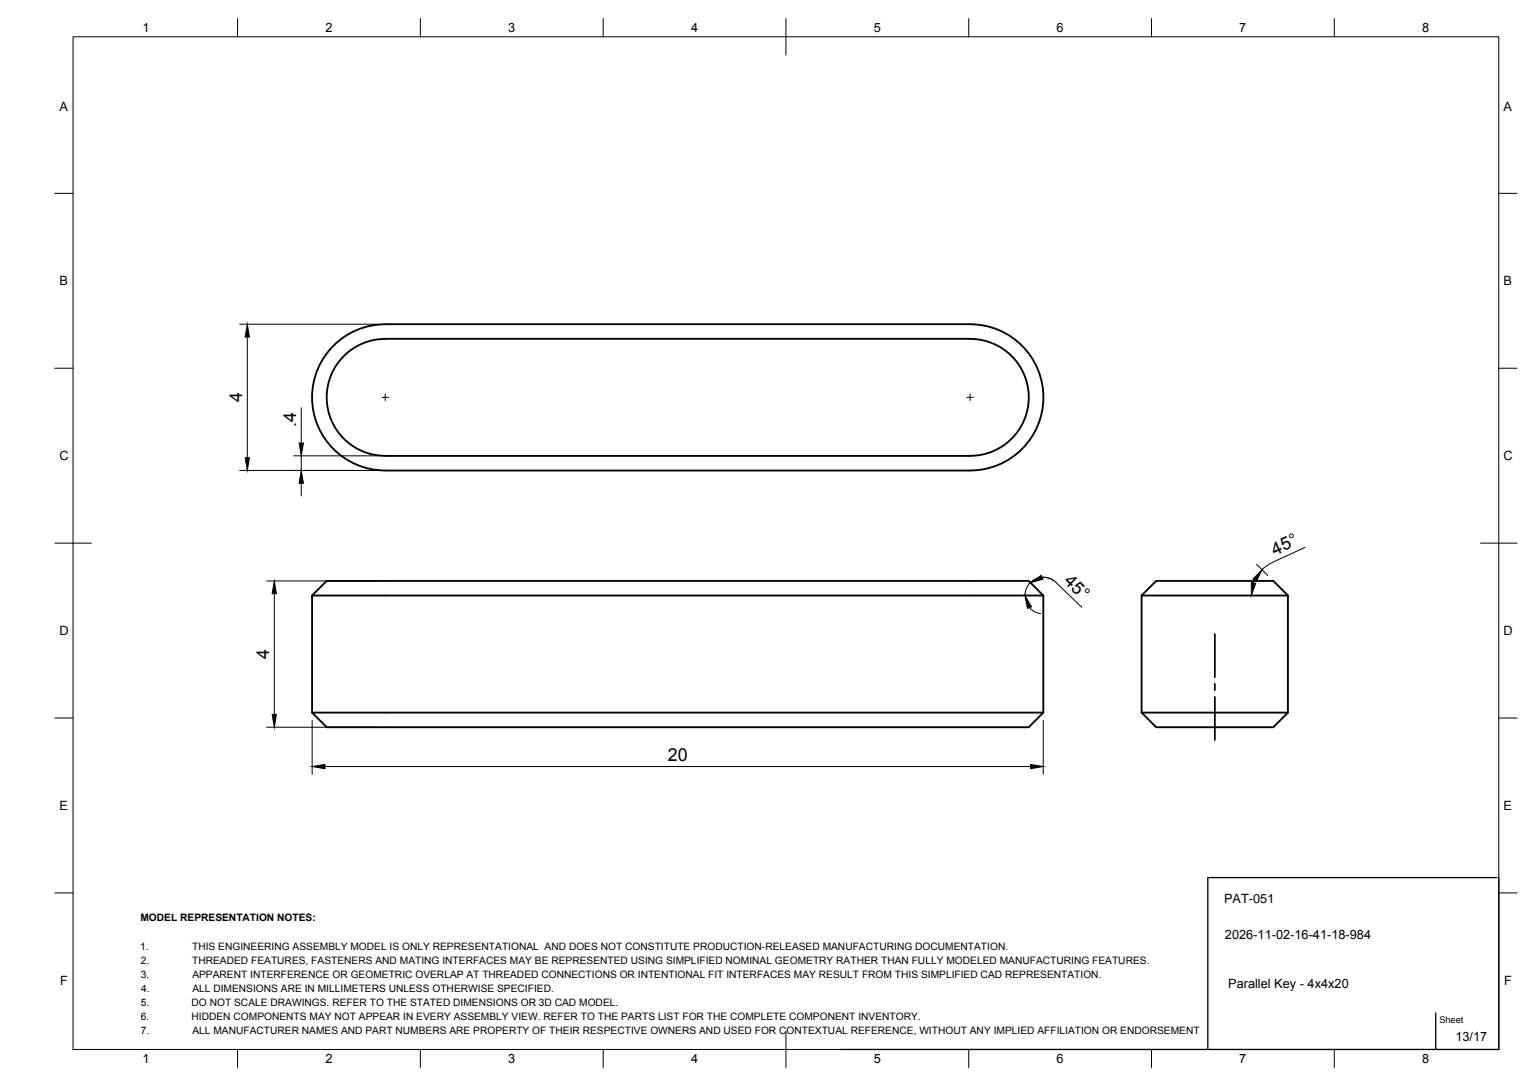
ISO-10303-21;
HEADER;
/* Generated by software containing ST-Developer
 * from STEP Tools, Inc. (www.steptools.com) 
 */

FILE_DESCRIPTION(
/* description */ ('Hand-crank flanged shaft unit'),
/* implementation_level */ '2;1');

FILE_NAME(
/* name */ 'Parallel Key - 4x4x20.step',
/* time_stamp */ '2026-10-27T18:35:45-07:00',
/* author */ (''),
/* organization */ (''),
/* preprocessor_version */ 'ST-DEVELOPER v20.2',
/* originating_system */ 'Autodesk Translation Framework v15.17.0.0',
/* authorisation */ '');

FILE_SCHEMA (('AUTOMOTIVE_DESIGN { 1 0 10303 214 3 1 1 }'));
ENDSEC;

DATA;
#10=MECHANICAL_DESIGN_GEOMETRIC_PRESENTATION_REPRESENTATION('',(#296),#6805);
#18=CONICAL_SURFACE('',#3857,0.18,0.785398163397448);
#19=CONICAL_SURFACE('',#3861,0.18,0.785398163397448);
#20=CONICAL_SURFACE('',#3869,0.18,0.785398163397449);
#21=CONICAL_SURFACE('',#3872,0.18,0.785398163397449);
#255=SHAPE_REPRESENTATION_RELATIONSHIP('SRR','None',#6918,#275);
#275=ADVANCED_BREP_SHAPE_REPRESENTATION('',(#316),#6801);
#296=STYLED_ITEM('',(#7091),#316);
#316=MANIFOLD_SOLID_BREP('Body1',#3338);
#487=PLANE('',#3856);
#488=PLANE('',#3860);
#489=PLANE('',#3866);
#490=PLANE('',#3867);
#491=PLANE('',#3868);
#492=PLANE('',#3871);
#493=PLANE('',#3876);
#494=PLANE('',#3877);
#658=FACE_OUTER_BOUND('',#930,.T.);
#659=FACE_OUTER_BOUND('',#931,.T.);
#660=FACE_OUTER_BOUND('',#932,.T.);
#661=FACE_OUTER_BOUND('',#933,.T.);
#662=FACE_OUTER_BOUND('',#934,.T.);
#663=FACE_OUTER_BOUND('',#935,.T.);
#664=FACE_OUTER_BOUND('',#936,.T.);
#665=FACE_OUTER_BOUND('',#937,.T.);
#666=FACE_OUTER_BOUND('',#938,.T.);
#667=FACE_OUTER_BOUND('',#939,.T.);
#668=FACE_OUTER_BOUND('',#940,.T.);
#669=FACE_OUTER_BOUND('',#941,.T.);
#670=FACE_OUTER_BOUND('',#942,.T.);
#671=FACE_OUTER_BOUND('',#943,.T.);
#930=EDGE_LOOP('',(#2885,#2886,#2887,#2888));
#931=EDGE_LOOP('',(#2889,#2890,#2891,#2892));
#932=EDGE_LOOP('',(#2893,#2894,#2895,#2896));
#933=EDGE_LOOP('',(#2897,#2898,#2899,#2900));
#934=EDGE_LOOP('',(#2901,#2902,#2903,#2904));
#935=EDGE_LOOP('',(#2905,#2906,#2907,#2908));
#936=EDGE_LOOP('',(#2909,#2910,#2911,#2912));
#937=EDGE_LOOP('',(#2913,#2914,#2915,#2916));
#938=EDGE_LOOP('',(#2917,#2918,#2919,#2920));
#939=EDGE_LOOP('',(#2921,#2922,#2923,#2924));
#940=EDGE_LOOP('',(#2925,#2926,#2927,#2928));
#941=EDGE_LOOP('',(#2929,#2930,#2931,#2932));
#942=EDGE_LOOP('',(#2933,#2934,#2935,#2936));
#943=EDGE_LOOP('',(#2937,#2938,#2939,#2940));
#1142=LINE('',#6488,#1370);
#1143=LINE('',#6490,#1371);
#1144=LINE('',#6492,#1372);
#1145=LINE('',#6493,#1373);
#1146=LINE('',#6497,#1374);
#1147=LINE('',#6503,#1375);
#1148=LINE('',#6504,#1376);
#1149=LINE('',#6505,#1377);
#1150=LINE('',#6511,#1378);
#1151=LINE('',#6514,#1379);
#1152=LINE('',#6517,#1380);
#1153=LINE('',#6518,#1381);
#1154=LINE('',#6522,#1382);
#1155=LINE('',#6524,#1383);
#1156=LINE('',#6525,#1384);
#1157=LINE('',#6528,#1385);
#1158=LINE('',#6533,#1386);
#1159=LINE('',#6534,#1387);
#1160=LINE('',#6535,#1388);
#1161=LINE('',#6540,#1389);
#1370=VECTOR('',#4707,1.);
#1371=VECTOR('',#4708,1.);
#1372=VECTOR('',#4709,1.);
#1373=VECTOR('',#4710,1.);
#1374=VECTOR('',#4713,1.);
#1375=VECTOR('',#4720,1.);
#1376=VECTOR('',#4721,1.);
#1377=VECTOR('',#4722,1.);
#1378=VECTOR('',#4731,1.);
#1379=VECTOR('',#4734,1.);
#1380=VECTOR('',#4737,1.);
#1381=VECTOR('',#4738,1.);
#1382=VECTOR('',#4743,1.);
#1383=VECTOR('',#4744,1.);
#1384=VECTOR('',#4745,1.);
#1385=VECTOR('',#4748,1.);
#1386=VECTOR('',#4753,1.);
#1387=VECTOR('',#4754,1.);
#1388=VECTOR('',#4755,1.);
#1389=VECTOR('',#4764,1.);
#1547=CIRCLE('',#3858,0.16);
#1548=CIRCLE('',#3859,0.2);
#1549=CIRCLE('',#3862,0.16);
#1550=CIRCLE('',#3863,0.2);
#1551=CIRCLE('',#3865,0.2);
#1552=CIRCLE('',#3870,0.16);
#1553=CIRCLE('',#3873,0.2);
#1554=CIRCLE('',#3874,0.16);
#1787=VERTEX_POINT('',#6486);
#1788=VERTEX_POINT('',#6487);
#1789=VERTEX_POINT('',#6489);
#1790=VERTEX_POINT('',#6491);
#1791=VERTEX_POINT('',#6495);
#1792=VERTEX_POINT('',#6496);
#1793=VERTEX_POINT('',#6501);
#1794=VERTEX_POINT('',#6502);
#1795=VERTEX_POINT('',#6510);
#1796=VERTEX_POINT('',#6512);
#1797=VERTEX_POINT('',#6516);
#1798=VERTEX_POINT('',#6521);
#1799=VERTEX_POINT('',#6523);
#1800=VERTEX_POINT('',#6527);
#1801=VERTEX_POINT('',#6531);
#1802=VERTEX_POINT('',#6532);
#2160=EDGE_CURVE('',#1787,#1788,#1142,.T.);
#2161=EDGE_CURVE('',#1788,#1789,#1143,.T.);
#2162=EDGE_CURVE('',#1789,#1790,#1144,.T.);
#2163=EDGE_CURVE('',#1790,#1787,#1145,.T.);
#2164=EDGE_CURVE('',#1791,#1792,#1146,.T.);
#2165=EDGE_CURVE('',#1792,#1788,#1547,.T.);
#2166=EDGE_CURVE('',#1787,#1791,#1548,.T.);
#2167=EDGE_CURVE('',#1793,#1794,#1147,.T.);
#2168=EDGE_CURVE('',#1794,#1792,#1148,.T.);
#2169=EDGE_CURVE('',#1791,#1793,#1149,.T.);
#2170=EDGE_CURVE('',#1789,#1794,#1549,.T.);
#2171=EDGE_CURVE('',#1793,#1790,#1550,.T.);
#2172=EDGE_CURVE('',#1795,#1787,#1150,.T.);
#2173=EDGE_CURVE('',#1796,#1795,#1551,.T.);
#2174=EDGE_CURVE('',#1796,#1791,#1151,.T.);
#2175=EDGE_CURVE('',#1797,#1790,#1152,.T.);
#2176=EDGE_CURVE('',#1795,#1797,#1153,.T.);
#2177=EDGE_CURVE('',#1798,#1795,#1154,.T.);
#2178=EDGE_CURVE('',#1797,#1799,#1155,.T.);
#2179=EDGE_CURVE('',#1799,#1798,#1156,.T.);
#2180=EDGE_CURVE('',#1800,#1796,#1157,.T.);
#2181=EDGE_CURVE('',#1798,#1800,#1552,.T.);
#2182=EDGE_CURVE('',#1801,#1802,#1158,.T.);
#2183=EDGE_CURVE('',#1802,#1796,#1159,.T.);
#2184=EDGE_CURVE('',#1800,#1801,#1160,.T.);
#2185=EDGE_CURVE('',#1797,#1802,#1553,.T.);
#2186=EDGE_CURVE('',#1801,#1799,#1554,.T.);
#2187=EDGE_CURVE('',#1802,#1793,#1161,.T.);
#2885=ORIENTED_EDGE('',*,*,#2160,.T.);
#2886=ORIENTED_EDGE('',*,*,#2161,.T.);
#2887=ORIENTED_EDGE('',*,*,#2162,.T.);
#2888=ORIENTED_EDGE('',*,*,#2163,.T.);
#2889=ORIENTED_EDGE('',*,*,#2164,.T.);
#2890=ORIENTED_EDGE('',*,*,#2165,.T.);
#2891=ORIENTED_EDGE('',*,*,#2160,.F.);
#2892=ORIENTED_EDGE('',*,*,#2166,.T.);
#2893=ORIENTED_EDGE('',*,*,#2167,.T.);
#2894=ORIENTED_EDGE('',*,*,#2168,.T.);
#2895=ORIENTED_EDGE('',*,*,#2164,.F.);
#2896=ORIENTED_EDGE('',*,*,#2169,.T.);
#2897=ORIENTED_EDGE('',*,*,#2162,.F.);
#2898=ORIENTED_EDGE('',*,*,#2170,.T.);
#2899=ORIENTED_EDGE('',*,*,#2167,.F.);
#2900=ORIENTED_EDGE('',*,*,#2171,.T.);
#2901=ORIENTED_EDGE('',*,*,#2166,.F.);
#2902=ORIENTED_EDGE('',*,*,#2172,.F.);
#2903=ORIENTED_EDGE('',*,*,#2173,.F.);
#2904=ORIENTED_EDGE('',*,*,#2174,.T.);
#2905=ORIENTED_EDGE('',*,*,#2163,.F.);
#2906=ORIENTED_EDGE('',*,*,#2175,.F.);
#2907=ORIENTED_EDGE('',*,*,#2176,.F.);
#2908=ORIENTED_EDGE('',*,*,#2172,.T.);
#2909=ORIENTED_EDGE('',*,*,#2161,.F.);
#2910=ORIENTED_EDGE('',*,*,#2165,.F.);
#2911=ORIENTED_EDGE('',*,*,#2168,.F.);
#2912=ORIENTED_EDGE('',*,*,#2170,.F.);
#2913=ORIENTED_EDGE('',*,*,#2177,.T.);
#2914=ORIENTED_EDGE('',*,*,#2176,.T.);
#2915=ORIENTED_EDGE('',*,*,#2178,.T.);
#2916=ORIENTED_EDGE('',*,*,#2179,.T.);
#2917=ORIENTED_EDGE('',*,*,#2180,.T.);
#2918=ORIENTED_EDGE('',*,*,#2173,.T.);
#2919=ORIENTED_EDGE('',*,*,#2177,.F.);
#2920=ORIENTED_EDGE('',*,*,#2181,.T.);
#2921=ORIENTED_EDGE('',*,*,#2182,.T.);
#2922=ORIENTED_EDGE('',*,*,#2183,.T.);
#2923=ORIENTED_EDGE('',*,*,#2180,.F.);
#2924=ORIENTED_EDGE('',*,*,#2184,.T.);
#2925=ORIENTED_EDGE('',*,*,#2178,.F.);
#2926=ORIENTED_EDGE('',*,*,#2185,.T.);
#2927=ORIENTED_EDGE('',*,*,#2182,.F.);
#2928=ORIENTED_EDGE('',*,*,#2186,.T.);
#2929=ORIENTED_EDGE('',*,*,#2171,.F.);
#2930=ORIENTED_EDGE('',*,*,#2187,.F.);
#2931=ORIENTED_EDGE('',*,*,#2185,.F.);
#2932=ORIENTED_EDGE('',*,*,#2175,.T.);
#2933=ORIENTED_EDGE('',*,*,#2179,.F.);
#2934=ORIENTED_EDGE('',*,*,#2186,.F.);
#2935=ORIENTED_EDGE('',*,*,#2184,.F.);
#2936=ORIENTED_EDGE('',*,*,#2181,.F.);
#2937=ORIENTED_EDGE('',*,*,#2169,.F.);
#2938=ORIENTED_EDGE('',*,*,#2174,.F.);
#2939=ORIENTED_EDGE('',*,*,#2183,.F.);
#2940=ORIENTED_EDGE('',*,*,#2187,.T.);
#3125=CYLINDRICAL_SURFACE('',#3864,0.2);
#3126=CYLINDRICAL_SURFACE('',#3875,0.2);
#3275=ADVANCED_FACE('',(#658),#487,.T.);
#3276=ADVANCED_FACE('',(#659),#18,.T.);
#3277=ADVANCED_FACE('',(#660),#488,.T.);
#3278=ADVANCED_FACE('',(#661),#19,.T.);
#3279=ADVANCED_FACE('',(#662),#3125,.T.);
#3280=ADVANCED_FACE('',(#663),#489,.T.);
#3281=ADVANCED_FACE('',(#664),#490,.T.);
#3282=ADVANCED_FACE('',(#665),#491,.T.);
#3283=ADVANCED_FACE('',(#666),#20,.T.);
#3284=ADVANCED_FACE('',(#667),#492,.T.);
#3285=ADVANCED_FACE('',(#668),#21,.T.);
#3286=ADVANCED_FACE('',(#669),#3126,.T.);
#3287=ADVANCED_FACE('',(#670),#493,.F.);
#3288=ADVANCED_FACE('',(#671),#494,.T.);
#3338=CLOSED_SHELL('',(#3275,#3276,#3277,#3278,#3279,#3280,#3281,#3282,
#3283,#3284,#3285,#3286,#3287,#3288));
#3855=AXIS2_PLACEMENT_3D('',#6484,#4703,#4704);
#3856=AXIS2_PLACEMENT_3D('',#6485,#4705,#4706);
#3857=AXIS2_PLACEMENT_3D('',#6494,#4711,#4712);
#3858=AXIS2_PLACEMENT_3D('',#6498,#4714,#4715);
#3859=AXIS2_PLACEMENT_3D('',#6499,#4716,#4717);
#3860=AXIS2_PLACEMENT_3D('',#6500,#4718,#4719);
#3861=AXIS2_PLACEMENT_3D('',#6506,#4723,#4724);
#3862=AXIS2_PLACEMENT_3D('',#6507,#4725,#4726);
#3863=AXIS2_PLACEMENT_3D('',#6508,#4727,#4728);
#3864=AXIS2_PLACEMENT_3D('',#6509,#4729,#4730);
#3865=AXIS2_PLACEMENT_3D('',#6513,#4732,#4733);
#3866=AXIS2_PLACEMENT_3D('',#6515,#4735,#4736);
#3867=AXIS2_PLACEMENT_3D('',#6519,#4739,#4740);
#3868=AXIS2_PLACEMENT_3D('',#6520,#4741,#4742);
#3869=AXIS2_PLACEMENT_3D('',#6526,#4746,#4747);
#3870=AXIS2_PLACEMENT_3D('',#6529,#4749,#4750);
#3871=AXIS2_PLACEMENT_3D('',#6530,#4751,#4752);
#3872=AXIS2_PLACEMENT_3D('',#6536,#4756,#4757);
#3873=AXIS2_PLACEMENT_3D('',#6537,#4758,#4759);
#3874=AXIS2_PLACEMENT_3D('',#6538,#4760,#4761);
#3875=AXIS2_PLACEMENT_3D('',#6539,#4762,#4763);
#3876=AXIS2_PLACEMENT_3D('',#6541,#4765,#4766);
#3877=AXIS2_PLACEMENT_3D('',#6542,#4767,#4768);
#4703=DIRECTION('axis',(0.,0.,1.));
#4704=DIRECTION('refdir',(1.,0.,0.));
#4705=DIRECTION('center_axis',(0.,0.707106781186548,0.707106781186547));
#4706=DIRECTION('ref_axis',(1.,0.,0.));
#4707=DIRECTION('',(-1.96261557335472E-15,-0.707106781186547,0.707106781186548));
#4708=DIRECTION('',(1.,0.,0.));
#4709=DIRECTION('',(0.,0.707106781186547,-0.707106781186548));
#4710=DIRECTION('',(-1.,0.,0.));
#4711=DIRECTION('center_axis',(0.,0.,-1.));
#4712=DIRECTION('ref_axis',(0.,1.,0.));
#4713=DIRECTION('',(0.,0.707106781186548,0.707106781186548));
#4714=DIRECTION('center_axis',(0.,0.,-1.));
#4715=DIRECTION('ref_axis',(0.,1.,0.));
#4716=DIRECTION('center_axis',(0.,0.,1.));
#4717=DIRECTION('ref_axis',(0.,1.,0.));
#4718=DIRECTION('center_axis',(0.,-0.707106781186548,0.707106781186547));
#4719=DIRECTION('ref_axis',(1.,0.,0.));
#4720=DIRECTION('',(1.96261557335472E-15,0.707106781186547,0.707106781186548));
#4721=DIRECTION('',(-1.,0.,0.));
#4722=DIRECTION('',(1.,0.,0.));
#4723=DIRECTION('center_axis',(0.,0.,-1.));
#4724=DIRECTION('ref_axis',(0.,-1.,0.));
#4725=DIRECTION('center_axis',(0.,0.,-1.));
#4726=DIRECTION('ref_axis',(0.,-1.,0.));
#4727=DIRECTION('center_axis',(0.,0.,1.));
#4728=DIRECTION('ref_axis',(0.,-1.,0.));
#4729=DIRECTION('center_axis',(0.,0.,1.));
#4730=DIRECTION('ref_axis',(0.,1.,0.));
#4731=DIRECTION('',(0.,0.,1.));
#4732=DIRECTION('center_axis',(0.,0.,-1.));
#4733=DIRECTION('ref_axis',(0.,1.,0.));
#4734=DIRECTION('',(0.,0.,1.));
#4735=DIRECTION('center_axis',(0.,1.,0.));
#4736=DIRECTION('ref_axis',(-1.,0.,0.));
#4737=DIRECTION('',(0.,0.,1.));
#4738=DIRECTION('',(1.,0.,0.));
#4739=DIRECTION('center_axis',(0.,0.,1.));
#4740=DIRECTION('ref_axis',(1.,0.,0.));
#4741=DIRECTION('center_axis',(0.,0.707106781186548,-0.707106781186548));
#4742=DIRECTION('ref_axis',(-1.,0.,0.));
#4743=DIRECTION('',(1.96261557335472E-15,0.707106781186548,0.707106781186548));
#4744=DIRECTION('',(0.,-0.707106781186548,-0.707106781186548));
#4745=DIRECTION('',(-1.,0.,0.));
#4746=DIRECTION('center_axis',(0.,0.,1.));
#4747=DIRECTION('ref_axis',(0.,1.,0.));
#4748=DIRECTION('',(0.,-0.707106781186548,0.707106781186547));
#4749=DIRECTION('center_axis',(0.,0.,1.));
#4750=DIRECTION('ref_axis',(0.,1.,0.));
#4751=DIRECTION('center_axis',(0.,-0.707106781186548,-0.707106781186548));
#4752=DIRECTION('ref_axis',(-1.,0.,0.));
#4753=DIRECTION('',(-1.96261557335472E-15,-0.707106781186548,0.707106781186548));
#4754=DIRECTION('',(-1.,0.,0.));
#4755=DIRECTION('',(1.,0.,0.));
#4756=DIRECTION('center_axis',(0.,0.,1.));
#4757=DIRECTION('ref_axis',(0.,-1.,0.));
#4758=DIRECTION('center_axis',(0.,0.,-1.));
#4759=DIRECTION('ref_axis',(0.,-1.,0.));
#4760=DIRECTION('center_axis',(0.,0.,1.));
#4761=DIRECTION('ref_axis',(0.,-1.,0.));
#4762=DIRECTION('center_axis',(0.,0.,1.));
#4763=DIRECTION('ref_axis',(0.,-1.,0.));
#4764=DIRECTION('',(0.,0.,1.));
#4765=DIRECTION('center_axis',(0.,0.,1.));
#4766=DIRECTION('ref_axis',(1.,0.,0.));
#4767=DIRECTION('center_axis',(0.,-1.,0.));
#4768=DIRECTION('ref_axis',(1.,0.,0.));
#6484=CARTESIAN_POINT('',(0.,0.,0.));
#6485=CARTESIAN_POINT('Origin',(0.4,0.18,0.38));
#6486=CARTESIAN_POINT('',(-0.8,0.2,0.36));
#6487=CARTESIAN_POINT('',(-0.8,0.16,0.4));
#6488=CARTESIAN_POINT('',(-0.8,0.2,0.36));
#6489=CARTESIAN_POINT('',(0.8,0.16,0.4));
#6490=CARTESIAN_POINT('',(0.4,0.16,0.4));
#6491=CARTESIAN_POINT('',(0.8,0.2,0.36));
#6492=CARTESIAN_POINT('',(0.8,0.16,0.4));
#6493=CARTESIAN_POINT('',(0.4,0.2,0.36));
#6494=CARTESIAN_POINT('Origin',(-0.8,0.,0.38));
#6495=CARTESIAN_POINT('',(-0.8,-0.2,0.36));
#6496=CARTESIAN_POINT('',(-0.8,-0.16,0.4));
#6497=CARTESIAN_POINT('',(-0.8,-0.2,0.36));
#6498=CARTESIAN_POINT('Origin',(-0.8,0.,0.4));
#6499=CARTESIAN_POINT('Origin',(-0.8,0.,0.36));
#6500=CARTESIAN_POINT('Origin',(-0.4,-0.18,0.38));
#6501=CARTESIAN_POINT('',(0.8,-0.2,0.36));
#6502=CARTESIAN_POINT('',(0.8,-0.16,0.4));
#6503=CARTESIAN_POINT('',(0.8,-0.2,0.36));
#6504=CARTESIAN_POINT('',(-0.4,-0.16,0.4));
#6505=CARTESIAN_POINT('',(-0.4,-0.2,0.36));
#6506=CARTESIAN_POINT('Origin',(0.8,0.,0.38));
#6507=CARTESIAN_POINT('Origin',(0.8,0.,0.4));
#6508=CARTESIAN_POINT('Origin',(0.8,0.,0.36));
#6509=CARTESIAN_POINT('Origin',(-0.8,0.,0.));
#6510=CARTESIAN_POINT('',(-0.8,0.2,0.04));
#6511=CARTESIAN_POINT('',(-0.8,0.2,0.));
#6512=CARTESIAN_POINT('',(-0.8,-0.2,0.04));
#6513=CARTESIAN_POINT('Origin',(-0.8,0.,0.04));
#6514=CARTESIAN_POINT('',(-0.8,-0.2,0.));
#6515=CARTESIAN_POINT('Origin',(0.8,0.2,0.));
#6516=CARTESIAN_POINT('',(0.8,0.2,0.04));
#6517=CARTESIAN_POINT('',(0.8,0.2,0.));
#6518=CARTESIAN_POINT('',(0.4,0.2,0.04));
#6519=CARTESIAN_POINT('Origin',(0.,0.,0.4));
#6520=CARTESIAN_POINT('Origin',(0.4,0.18,0.02));
#6521=CARTESIAN_POINT('',(-0.8,0.16,0.));
#6522=CARTESIAN_POINT('',(-0.8,0.16,0.));
#6523=CARTESIAN_POINT('',(0.8,0.16,0.));
#6524=CARTESIAN_POINT('',(0.8,0.2,0.04));
#6525=CARTESIAN_POINT('',(0.4,0.16,0.));
#6526=CARTESIAN_POINT('Origin',(-0.8,0.,0.02));
#6527=CARTESIAN_POINT('',(-0.8,-0.16,0.));
#6528=CARTESIAN_POINT('',(-0.8,-0.16,0.));
#6529=CARTESIAN_POINT('Origin',(-0.8,0.,0.));
#6530=CARTESIAN_POINT('Origin',(-0.4,-0.18,0.02));
#6531=CARTESIAN_POINT('',(0.8,-0.16,0.));
#6532=CARTESIAN_POINT('',(0.8,-0.2,0.04));
#6533=CARTESIAN_POINT('',(0.8,-0.16,0.));
#6534=CARTESIAN_POINT('',(-0.4,-0.2,0.04));
#6535=CARTESIAN_POINT('',(-0.4,-0.16,0.));
#6536=CARTESIAN_POINT('Origin',(0.8,0.,0.02));
#6537=CARTESIAN_POINT('Origin',(0.8,0.,0.04));
#6538=CARTESIAN_POINT('Origin',(0.8,0.,0.));
#6539=CARTESIAN_POINT('Origin',(0.8,0.,0.));
#6540=CARTESIAN_POINT('',(0.8,-0.2,0.));
#6541=CARTESIAN_POINT('Origin',(0.,0.,0.));
#6542=CARTESIAN_POINT('Origin',(-0.8,-0.2,0.));
#6776=UNCERTAINTY_MEASURE_WITH_UNIT(LENGTH_MEASURE(0.001),#6806,
'DISTANCE_ACCURACY_VALUE',
'Maximum model space distance between geometric entities at asserted c
onnectivities');
#6780=UNCERTAINTY_MEASURE_WITH_UNIT(LENGTH_MEASURE(0.001),#6806,
'DISTANCE_ACCURACY_VALUE',
'Maximum model space distance between geometric entities at asserted c
onnectivities');
#6801=(
GEOMETRIC_REPRESENTATION_CONTEXT(3)
GLOBAL_UNCERTAINTY_ASSIGNED_CONTEXT((#6776))
GLOBAL_UNIT_ASSIGNED_CONTEXT((#6806,#6808,#6809))
REPRESENTATION_CONTEXT('','3D')
);
#6805=(
GEOMETRIC_REPRESENTATION_CONTEXT(3)
GLOBAL_UNCERTAINTY_ASSIGNED_CONTEXT((#6780))
GLOBAL_UNIT_ASSIGNED_CONTEXT((#6806,#6808,#6809))
REPRESENTATION_CONTEXT('','3D')
);
#6806=(
LENGTH_UNIT()
NAMED_UNIT(*)
SI_UNIT(.CENTI.,.METRE.)
);
#6808=(
NAMED_UNIT(*)
PLANE_ANGLE_UNIT()
SI_UNIT($,.RADIAN.)
);
#6809=(
NAMED_UNIT(*)
SI_UNIT($,.STERADIAN.)
SOLID_ANGLE_UNIT()
);
#6830=SHAPE_DEFINITION_REPRESENTATION(#6884,#6918);
#6884=PRODUCT_DEFINITION_SHAPE('',$,#6943);
#6918=SHAPE_REPRESENTATION('',(#3855),#6801);
#6922=PRODUCT_DEFINITION_CONTEXT('part definition',#6996,'design');
#6943=PRODUCT_DEFINITION('Parallel Key - 4x4x20',
'Parallel Key - 4x4x20',#6967,#6922);
#6967=PRODUCT_DEFINITION_FORMATION('',$,#7018);
#6996=APPLICATION_CONTEXT(
'Core Data for Automotive Mechanical Design Process');
#6997=PRODUCT_CONTEXT('part definition',#6996,'mechanical');
#7018=PRODUCT('Parallel Key - 4x4x20','Parallel Key - 4x4x20',
'Parallel Key - 4x4x20',(#6997));
#7085=COLOUR_RGB('Grey',0.48,0.52,0.57);
#7086=FILL_AREA_STYLE_COLOUR('',#7085);
#7087=FILL_AREA_STYLE('',(#7086));
#7088=SURFACE_STYLE_FILL_AREA(#7087);
#7089=SURFACE_SIDE_STYLE('',(#7088));
#7090=SURFACE_STYLE_USAGE(.BOTH.,#7089);
#7091=PRESENTATION_STYLE_ASSIGNMENT((#7090));
ENDSEC;
END-ISO-10303-21;
